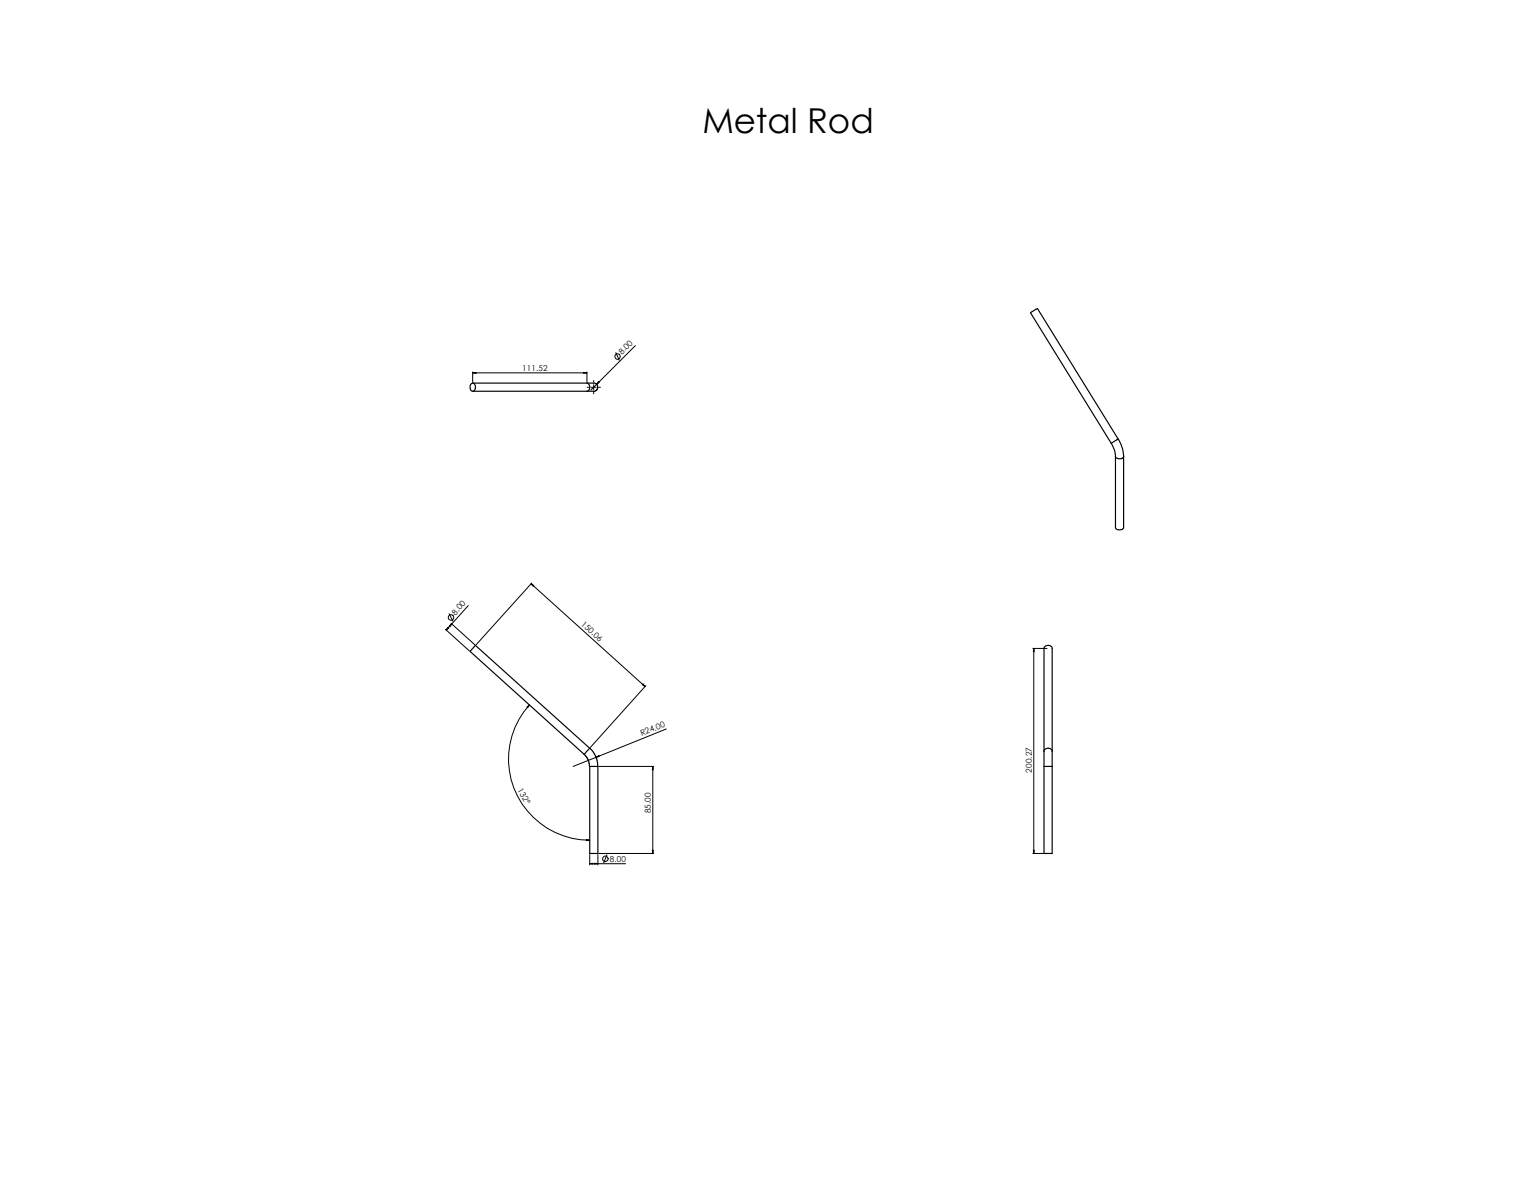
ISO-10303-21;
HEADER;
FILE_DESCRIPTION (('STEP AP214'),
    '1' );
FILE_NAME ('Metal Rod.step',
    '2026-10-20T14:49:59',
    ( '' ),
    ( '' ),
    'SwSTEP 2.0',
    'SolidWorks 2025',
    '' );
FILE_SCHEMA (( 'AUTOMOTIVE_DESIGN' ));
ENDSEC;

DATA;
#54=AXIS2_PLACEMENT_3D ( 'NONE', #4576, #604, #662 ) ;
#117=( NAMED_UNIT ( * ) SI_UNIT ( $, .STERADIAN. ) SOLID_ANGLE_UNIT ( ) );
#133=ADVANCED_BREP_SHAPE_REPRESENTATION ( '', ( #10321, #4601 ), #2278 ) ;
#147=SHAPE_REPRESENTATION_RELATIONSHIP ( 'NONE' , 'NONE' ,  #7587, #133 ) ;
#173=DIRECTION ( 'NONE',  ( 1.000000000000000000, 0.000000000000000000, 0.000000000000000000 ) ) ;
#205=CARTESIAN_POINT ( 'NONE',  ( -47.94539818030328604, 85.52895752738115220, 4.000000000000000000 ) ) ;
#218=VECTOR ( 'NONE', #1908, 1000.000000000000000 ) ;
#318=DIRECTION ( 'NONE',  ( 0.7431448254773962425, -0.6691306063588559061, 0.000000000000000000 ) ) ;
#324=DIRECTION ( 'NONE',  ( 6.106226635438360972E-16, -1.000000000000000000, 0.000000000000000000 ) ) ;
#334=ORIENTED_EDGE ( 'NONE', *, *, #6698, .T. ) ;
#338=CIRCLE ( 'NONE', #9475, 4.000000000000003553 ) ;
#367=DIRECTION ( 'NONE',  ( 1.000000000000000000, 0.000000000000000000, 0.000000000000000000 ) ) ;
#487=ADVANCED_FACE ( 'NONE', ( #1284 ), #6851, .T. ) ;
#497=CARTESIAN_POINT ( 'NONE',  ( -166.0794662972351716, 270.8019239353934040, 0.000000000000000000 ) ) ;
#536=ORIENTED_EDGE ( 'NONE', *, *, #7617, .T. ) ;
#601=CARTESIAN_POINT ( 'NONE',  ( -47.94539818030328604, 70.52895752738115220, 0.000000000000000000 ) ) ;
#604=DIRECTION ( 'NONE',  ( 0.000000000000000000, 0.000000000000000000, 1.000000000000000000 ) ) ;
#662=DIRECTION ( 'NONE',  ( 1.000000000000000000, 0.000000000000000000, 0.000000000000000000 ) ) ;
#682=CARTESIAN_POINT ( 'NONE',  ( -47.94539818030328604, 70.52895752738115220, -4.000000000000000000 ) ) ;
#741=ORIENTED_EDGE ( 'NONE', *, *, #7129, .T. ) ;
#749=CARTESIAN_POINT ( 'NONE',  ( -51.88626362769068123, 173.3644333388386940, 4.898587196589412829E-16 ) ) ;
#849=CARTESIAN_POINT ( 'NONE',  ( -166.0794662972351716, 270.8019239353934040, 0.000000000000000000 ) ) ;
#903=( NAMED_UNIT ( * ) PLANE_ANGLE_UNIT ( ) SI_UNIT ( $, .RADIAN. ) );
#922=DIRECTION ( 'NONE',  ( 0.000000000000000000, 1.000000000000000000, 0.000000000000000000 ) ) ;
#956=LINE ( 'NONE', #5088, #218 ) ;
#998=DIRECTION ( 'NONE',  ( 6.106226635438360972E-16, -1.000000000000000000, 0.000000000000000000 ) ) ;
#1070=DIRECTION ( 'NONE',  ( 1.000000000000000000, 0.000000000000000000, 0.000000000000000000 ) ) ;
#1154=DIRECTION ( 'NONE',  ( 0.000000000000000000, 1.000000000000000000, 0.000000000000000000 ) ) ;
#1284=FACE_OUTER_BOUND ( 'NONE', #3777, .T. ) ;
#1395=EDGE_CURVE ( 'NONE', #9655, #10447, #7716, .T. ) ;
#1528=DIRECTION ( 'NONE',  ( 1.000000000000000000, 0.000000000000000000, 0.000000000000000000 ) ) ;
#1635=AXIS2_PLACEMENT_3D ( 'NONE', #2392, #3294, #6585 ) ;
#1662=ORIENTED_EDGE ( 'NONE', *, *, #7675, .T. ) ;
#1863=CARTESIAN_POINT ( 'NONE',  ( -166.0794662972351716, 270.8019239353934040, 0.000000000000000000 ) ) ;
#1881=CIRCLE ( 'NONE', #54, 24.00000000000002132 ) ;
#1889=VERTEX_POINT ( 'NONE', #3894 ) ;
#1908=DIRECTION ( 'NONE',  ( -0.7431448254773957984, 0.6691306063588564612, 0.000000000000000000 ) ) ;
#1946=ORIENTED_EDGE ( 'NONE', *, *, #10327, .F. ) ;
#1950=DIRECTION ( 'NONE',  ( 1.000000000000000000, 6.106226635438360972E-16, 0.000000000000000000 ) ) ;
#2124=PRODUCT_DEFINITION_SHAPE ( 'NONE', 'NONE',  #3203 ) ;
#2211=DIRECTION ( 'NONE',  ( 0.7431448254773962425, -0.6691306063588559061, 0.000000000000000000 ) ) ;
#2214=CARTESIAN_POINT ( 'NONE',  ( -67.94539818030330025, 155.5289575273812090, 0.000000000000000000 ) ) ;
#2247=EDGE_CURVE ( 'NONE', #10447, #4228, #7356, .T. ) ;
#2278=( GEOMETRIC_REPRESENTATION_CONTEXT ( 3 ) GLOBAL_UNCERTAINTY_ASSIGNED_CONTEXT ( ( #3360 ) ) GLOBAL_UNIT_ASSIGNED_CONTEXT ( ( #7398, #6601, #9089 ) ) REPRESENTATION_CONTEXT ( 'NONE', 'WORKASPACE' ) );
#2317=AXIS2_PLACEMENT_3D ( 'NONE', #6483, #922, #7389 ) ;
#2320=ADVANCED_FACE ( 'NONE', ( #6609 ), #8357, .T. ) ;
#2340=EDGE_CURVE ( 'NONE', #10187, #1889, #5692, .T. ) ;
#2365=ORIENTED_EDGE ( 'NONE', *, *, #5529, .F. ) ;
#2392=CARTESIAN_POINT ( 'NONE',  ( -47.94539818030328604, 155.5289575273811522, 0.000000000000000000 ) ) ;
#2414=EDGE_CURVE ( 'NONE', #9655, #4137, #10114, .T. ) ;
#2441=DIRECTION ( 'NONE',  ( 0.6691306063588561281, 0.7431448254773961315, 0.000000000000000000 ) ) ;
#2460=ORIENTED_EDGE ( 'NONE', *, *, #2340, .F. ) ;
#2493=DIRECTION ( 'NONE',  ( 0.7431448254773962425, -0.6691306063588559061, 0.000000000000000000 ) ) ;
#2502=AXIS2_PLACEMENT_3D ( 'NONE', #7643, #3779, #4518 ) ;
#2585=CARTESIAN_POINT ( 'NONE',  ( -54.56278605312611774, 170.3918540369290895, 0.000000000000000000 ) ) ;
#2637=ORIENTED_EDGE ( 'NONE', *, *, #6913, .F. ) ;
#2676=ORIENTED_EDGE ( 'NONE', *, *, #7129, .F. ) ;
#2688=DIRECTION ( 'NONE',  ( -0.6691306063588561281, -0.7431448254773961315, 0.000000000000000000 ) ) ;
#2717=ORIENTED_EDGE ( 'NONE', *, *, #2340, .T. ) ;
#2745=AXIS2_PLACEMENT_3D ( 'NONE', #8570, #2211, #7779 ) ;
#2758=ORIENTED_EDGE ( 'NONE', *, *, #6627, .T. ) ;
#2982=PLANE ( 'NONE',  #3774 ) ;
#2997=AXIS2_PLACEMENT_3D ( 'NONE', #4334, #9858, #2688 ) ;
#3039=ORIENTED_EDGE ( 'NONE', *, *, #5529, .T. ) ;
#3095=CIRCLE ( 'NONE', #3428, 16.00000000000001421 ) ;
#3109=EDGE_CURVE ( 'NONE', #4228, #9114, #338, .T. ) ;
#3203=PRODUCT_DEFINITION ( 'UNKNOWN', '', #7860, #5677 ) ;
#3226=CARTESIAN_POINT ( 'NONE',  ( -47.94539818030328604, 155.5289575273811522, 4.000000000000000000 ) ) ;
#3234=( LENGTH_UNIT ( ) NAMED_UNIT ( * ) SI_UNIT ( .MILLI., .METRE. ) );
#3294=DIRECTION ( 'NONE',  ( 6.106226635438360972E-16, -1.000000000000000000, 0.000000000000000000 ) ) ;
#3360=UNCERTAINTY_MEASURE_WITH_UNIT (LENGTH_MEASURE( 1.000000000000000082E-05 ), #7398, 'distance_accuracy_value', 'NONE');
#3416=STYLED_ITEM('',(#10518),#10321);
#3422=CIRCLE ( 'NONE', #2745, 3.999999999999998668 ) ;
#3428=AXIS2_PLACEMENT_3D ( 'NONE', #9716, #7072, #9621 ) ;
#3444=ORIENTED_EDGE ( 'NONE', *, *, #2247, .F. ) ;
#3531=ORIENTED_EDGE ( 'NONE', *, *, #10340, .F. ) ;
#3546=CARTESIAN_POINT ( 'NONE',  ( -47.94539818030328604, 70.52895752738115220, 0.000000000000000000 ) ) ;
#3607=AXIS2_PLACEMENT_3D ( 'NONE', #9456, #5362, #5417 ) ;
#3700=CARTESIAN_POINT ( 'NONE',  ( -47.94539818030328604, 85.52895752738115220, -4.000000000000000000 ) ) ;
#3774=AXIS2_PLACEMENT_3D ( 'NONE', #497, #9346, #7859 ) ;
#3777=EDGE_LOOP ( 'NONE', ( #9685, #6029, #7830, #3039, #3444 ) ) ;
#3779=DIRECTION ( 'NONE',  ( 0.000000000000000000, 1.000000000000000000, 0.000000000000000000 ) ) ;
#3828=PRODUCT ( 'Metal Rod', 'Metal Rod', '', ( #10421 ) ) ;
#3851=VECTOR ( 'NONE', #1154, 1000.000000000000000 ) ;
#3894=CARTESIAN_POINT ( 'NONE',  ( -57.23930847856152582, 167.4192747350194850, 0.000000000000000000 ) ) ;
#3942=DIRECTION ( 'NONE',  ( 1.000000000000000000, 0.000000000000000000, 0.000000000000000000 ) ) ;
#4009=AXIS2_PLACEMENT_3D ( 'NONE', #1863, #5092, #8326 ) ;
#4111=TOROIDAL_SURFACE ( 'NONE', #3607, 20.00000000000001776, 4.000000000000000000 ) ;
#4137=VERTEX_POINT ( 'NONE', #4611 ) ;
#4149=AXIS2_PLACEMENT_3D ( 'NONE', #8366, #324, #1950 ) ;
#4228=VERTEX_POINT ( 'NONE', #3226 ) ;
#4312=CARTESIAN_POINT ( 'NONE',  ( -51.94539818030329315, 155.5289575273811522, -4.898587196589407898E-16 ) ) ;
#4334=CARTESIAN_POINT ( 'NONE',  ( -54.56278605312608931, 170.3918540369290895, 0.000000000000000000 ) ) ;
#4397=PLANE ( 'NONE',  #4149 ) ;
#4414=ADVANCED_FACE ( 'NONE', ( #8574 ), #4397, .T. ) ;
#4518=DIRECTION ( 'NONE',  ( 0.000000000000000000, 0.000000000000000000, 1.000000000000000000 ) ) ;
#4576=CARTESIAN_POINT ( 'NONE',  ( -67.94539818030330025, 155.5289575273812090, 0.000000000000000000 ) ) ;
#4601=AXIS2_PLACEMENT_3D ( 'NONE', #8586, #5983, #5928 ) ;
#4611=CARTESIAN_POINT ( 'NONE',  ( -47.94539818030328604, 155.5289575273811522, -4.000000000000000000 ) ) ;
#4614=ORIENTED_EDGE ( 'NONE', *, *, #10327, .T. ) ;
#4628=APPLICATION_CONTEXT ( 'automotive_design' ) ;
#4763=CIRCLE ( 'NONE', #5613, 4.000000000000003553 ) ;
#4815=ADVANCED_FACE ( 'NONE', ( #8137 ), #7349, .T. ) ;
#4891=CYLINDRICAL_SURFACE ( 'NONE', #2317, 4.000000000000000000 ) ;
#4931=ORIENTED_EDGE ( 'NONE', *, *, #7675, .F. ) ;
#5088=CARTESIAN_POINT ( 'NONE',  ( -57.23930847856151161, 167.4192747350194850, 0.000000000000000000 ) ) ;
#5092=DIRECTION ( 'NONE',  ( 0.7431448254773962425, -0.6691306063588559061, 0.000000000000000000 ) ) ;
#5094=DIRECTION ( 'NONE',  ( 6.106226635438360972E-16, -1.000000000000000000, 0.000000000000000000 ) ) ;
#5107=APPLICATION_CONTEXT ( 'automotive_design' ) ;
#5166=DIRECTION ( 'NONE',  ( -0.6691306063588561281, -0.7431448254773961315, 0.000000000000000000 ) ) ;
#5190=ADVANCED_FACE ( 'NONE', ( #9680 ), #4891, .T. ) ;
#5209=FACE_OUTER_BOUND ( 'NONE', #9931, .T. ) ;
#5210=CARTESIAN_POINT ( 'NONE',  ( -168.7559887226705655, 267.8293446334838563, 0.000000000000000000 ) ) ;
#5223=CARTESIAN_POINT ( 'NONE',  ( -54.56278605312608931, 170.3918540369290895, 0.000000000000000000 ) ) ;
#5302=VERTEX_POINT ( 'NONE', #5210 ) ;
#5362=DIRECTION ( 'NONE',  ( 0.000000000000000000, 0.000000000000000000, 1.000000000000000000 ) ) ;
#5368=CLOSED_SHELL ( 'NONE', ( #7444, #2320, #487, #4815, #8507, #5190, #7409, #4414 ) ) ;
#5412=ORIENTED_EDGE ( 'NONE', *, *, #6698, .F. ) ;
#5417=DIRECTION ( 'NONE',  ( 1.000000000000000000, 0.000000000000000000, 0.000000000000000000 ) ) ;
#5420=CARTESIAN_POINT ( 'NONE',  ( -51.88626362769066702, 173.3644333388386656, 4.898587196589412829E-16 ) ) ;
#5529=EDGE_CURVE ( 'NONE', #9125, #4228, #10282, .T. ) ;
#5613=AXIS2_PLACEMENT_3D ( 'NONE', #7428, #7474, #173 ) ;
#5657=CARTESIAN_POINT ( 'NONE',  ( -47.94539818030328604, 155.5289575273811522, 0.000000000000000000 ) ) ;
#5677=PRODUCT_DEFINITION_CONTEXT ( 'detailed design', #5107, 'design' ) ;
#5692=CIRCLE ( 'NONE', #6375, 3.999999999999998668 ) ;
#5725=EDGE_CURVE ( 'NONE', #9869, #5302, #8575, .T. ) ;
#5741=SHAPE_DEFINITION_REPRESENTATION ( #2124, #7587 ) ;
#5781=UNCERTAINTY_MEASURE_WITH_UNIT (LENGTH_MEASURE( 1.000000000000000082E-05 ), #3234, 'distance_accuracy_value', 'NONE');
#5888=CARTESIAN_POINT ( 'NONE',  ( -47.94539818030328604, 155.5289575273811522, 0.000000000000000000 ) ) ;
#5928=DIRECTION ( 'NONE',  ( 1.000000000000000000, 0.000000000000000000, 0.000000000000000000 ) ) ;
#5983=DIRECTION ( 'NONE',  ( 0.000000000000000000, 0.000000000000000000, 1.000000000000000000 ) ) ;
#6015=AXIS2_PLACEMENT_3D ( 'NONE', #3546, #6770, #367 ) ;
#6029=ORIENTED_EDGE ( 'NONE', *, *, #2414, .T. ) ;
#6153=ORIENTED_EDGE ( 'NONE', *, *, #6627, .F. ) ;
#6161=EDGE_LOOP ( 'NONE', ( #2460, #334, #7393, #4931 ) ) ;
#6296=AXIS2_PLACEMENT_3D ( 'NONE', #849, #2493, #2441 ) ;
#6329=EDGE_LOOP ( 'NONE', ( #5412, #2676, #1662, #6904 ) ) ;
#6334=AXIS2_PLACEMENT_3D ( 'NONE', #2214, #10227, #1528 ) ;
#6374=LINE ( 'NONE', #5420, #9686 ) ;
#6375=AXIS2_PLACEMENT_3D ( 'NONE', #2585, #318, #9103 ) ;
#6464=ORIENTED_EDGE ( 'NONE', *, *, #7617, .F. ) ;
#6483=CARTESIAN_POINT ( 'NONE',  ( -47.94539818030328604, 85.52895752738115220, 0.000000000000000000 ) ) ;
#6585=DIRECTION ( 'NONE',  ( 1.000000000000000000, 0.000000000000000000, 0.000000000000000000 ) ) ;
#6601=( NAMED_UNIT ( * ) PLANE_ANGLE_UNIT ( ) SI_UNIT ( $, .RADIAN. ) );
#6609=FACE_OUTER_BOUND ( 'NONE', #6161, .T. ) ;
#6624=AXIS2_PLACEMENT_3D ( 'NONE', #5657, #998, #8146 ) ;
#6627=EDGE_CURVE ( 'NONE', #9125, #10187, #1881, .T. ) ;
#6698=EDGE_CURVE ( 'NONE', #10187, #9869, #6374, .T. ) ;
#6717=VECTOR ( 'NONE', #8996, 1000.000000000000000 ) ;
#6770=DIRECTION ( 'NONE',  ( 6.106226635438360972E-16, -1.000000000000000000, 0.000000000000000000 ) ) ;
#6851=CYLINDRICAL_SURFACE ( 'NONE', #2502, 4.000000000000000000 ) ;
#6863=AXIS2_PLACEMENT_3D ( 'NONE', #5223, #8506, #5166 ) ;
#6904=ORIENTED_EDGE ( 'NONE', *, *, #10340, .T. ) ;
#6913=EDGE_CURVE ( 'NONE', #4137, #9125, #7143, .T. ) ;
#6973=MECHANICAL_DESIGN_GEOMETRIC_PRESENTATION_REPRESENTATION('',(#3416),#9687);
#7072=DIRECTION ( 'NONE',  ( 0.000000000000000000, 0.000000000000000000, 1.000000000000000000 ) ) ;
#7129=EDGE_CURVE ( 'NONE', #1889, #10187, #3422, .T. ) ;
#7143=CIRCLE ( 'NONE', #6624, 4.000000000000003553 ) ;
#7156=ORIENTED_EDGE ( 'NONE', *, *, #5725, .F. ) ;
#7243=ORIENTED_EDGE ( 'NONE', *, *, #2414, .F. ) ;
#7349=CYLINDRICAL_SURFACE ( 'NONE', #6863, 3.999999999999998668 ) ;
#7356=LINE ( 'NONE', #205, #6717 ) ;
#7389=DIRECTION ( 'NONE',  ( 0.000000000000000000, 0.000000000000000000, 1.000000000000000000 ) ) ;
#7393=ORIENTED_EDGE ( 'NONE', *, *, #5725, .T. ) ;
#7398=( LENGTH_UNIT ( ) NAMED_UNIT ( * ) SI_UNIT ( .MILLI., .METRE. ) );
#7409=ADVANCED_FACE ( 'NONE', ( #9296 ), #2982, .F. ) ;
#7428=CARTESIAN_POINT ( 'NONE',  ( -47.94539818030328604, 155.5289575273811522, 0.000000000000000000 ) ) ;
#7444=ADVANCED_FACE ( 'NONE', ( #5209 ), #4111, .T. ) ;
#7449=ORIENTED_EDGE ( 'NONE', *, *, #3109, .T. ) ;
#7474=DIRECTION ( 'NONE',  ( 6.106226635438360972E-16, -1.000000000000000000, 0.000000000000000000 ) ) ;
#7476=CIRCLE ( 'NONE', #6296, 3.999999999999998668 ) ;
#7538=EDGE_CURVE ( 'NONE', #10447, #9655, #10207, .T. ) ;
#7587=SHAPE_REPRESENTATION ( 'Metal Rod', ( #4601 ), #2278 ) ;
#7617=EDGE_CURVE ( 'NONE', #9114, #1889, #3095, .T. ) ;
#7643=CARTESIAN_POINT ( 'NONE',  ( -47.94539818030328604, 85.52895752738115220, 0.000000000000000000 ) ) ;
#7675=EDGE_CURVE ( 'NONE', #1889, #5302, #956, .T. ) ;
#7688=CARTESIAN_POINT ( 'NONE',  ( -47.94539818030328604, 70.52895752738115220, 4.000000000000000000 ) ) ;
#7694=EDGE_LOOP ( 'NONE', ( #3531, #7156 ) ) ;
#7716=CIRCLE ( 'NONE', #6015, 4.000000000000003553 ) ;
#7745=CARTESIAN_POINT ( 'NONE',  ( -43.94539818030328604, 155.5289575273811522, 0.000000000000000000 ) ) ;
#7779=DIRECTION ( 'NONE',  ( 0.6691306063588561281, 0.7431448254773961315, 0.000000000000000000 ) ) ;
#7830=ORIENTED_EDGE ( 'NONE', *, *, #6913, .T. ) ;
#7859=DIRECTION ( 'NONE',  ( 0.6691306063588559061, 0.7431448254773963535, 0.000000000000000000 ) ) ;
#7860=PRODUCT_DEFINITION_FORMATION_WITH_SPECIFIED_SOURCE ( 'ANY', '', #3828, .NOT_KNOWN. ) ;
#8137=FACE_OUTER_BOUND ( 'NONE', #6329, .T. ) ;
#8146=DIRECTION ( 'NONE',  ( 1.000000000000000000, 0.000000000000000000, 0.000000000000000000 ) ) ;
#8157=ORIENTED_EDGE ( 'NONE', *, *, #7538, .F. ) ;
#8326=DIRECTION ( 'NONE',  ( 0.6691306063588561281, 0.7431448254773961315, 0.000000000000000000 ) ) ;
#8357=CYLINDRICAL_SURFACE ( 'NONE', #2997, 3.999999999999998668 ) ;
#8366=CARTESIAN_POINT ( 'NONE',  ( -47.94539818030327893, 70.52895752738115220, 0.000000000000000000 ) ) ;
#8472=EDGE_LOOP ( 'NONE', ( #10160, #8804 ) ) ;
#8506=DIRECTION ( 'NONE',  ( -0.7431448254773957984, 0.6691306063588564612, 0.000000000000000000 ) ) ;
#8507=ADVANCED_FACE ( 'NONE', ( #9429 ), #8866, .T. ) ;
#8509=CARTESIAN_POINT ( 'NONE',  ( -163.4029438717997209, 273.7745032373030085, 4.898587196589412829E-16 ) ) ;
#8570=CARTESIAN_POINT ( 'NONE',  ( -54.56278605312611774, 170.3918540369290895, 0.000000000000000000 ) ) ;
#8574=FACE_OUTER_BOUND ( 'NONE', #8472, .T. ) ;
#8575=CIRCLE ( 'NONE', #4009, 3.999999999999998668 ) ;
#8586=CARTESIAN_POINT ( 'NONE',  ( 0.000000000000000000, 0.000000000000000000, 0.000000000000000000 ) ) ;
#8606=DIRECTION ( 'NONE',  ( -0.7431448254773957984, 0.6691306063588564612, 0.000000000000000000 ) ) ;
#8760=DIRECTION ( 'NONE',  ( 6.106226635438360972E-16, -1.000000000000000000, 0.000000000000000000 ) ) ;
#8804=ORIENTED_EDGE ( 'NONE', *, *, #1395, .T. ) ;
#8866=TOROIDAL_SURFACE ( 'NONE', #6334, 20.00000000000001776, 4.000000000000000000 ) ;
#8996=DIRECTION ( 'NONE',  ( 0.000000000000000000, 1.000000000000000000, 0.000000000000000000 ) ) ;
#9089=( NAMED_UNIT ( * ) SI_UNIT ( $, .STERADIAN. ) SOLID_ANGLE_UNIT ( ) );
#9103=DIRECTION ( 'NONE',  ( 0.6691306063588561281, 0.7431448254773961315, 0.000000000000000000 ) ) ;
#9114=VERTEX_POINT ( 'NONE', #4312 ) ;
#9125=VERTEX_POINT ( 'NONE', #7745 ) ;
#9296=FACE_OUTER_BOUND ( 'NONE', #7694, .T. ) ;
#9346=DIRECTION ( 'NONE',  ( 0.7431448254773963535, -0.6691306063588559061, 0.000000000000000000 ) ) ;
#9429=FACE_OUTER_BOUND ( 'NONE', #10316, .T. ) ;
#9456=CARTESIAN_POINT ( 'NONE',  ( -67.94539818030330025, 155.5289575273812090, 0.000000000000000000 ) ) ;
#9475=AXIS2_PLACEMENT_3D ( 'NONE', #5888, #5094, #1070 ) ;
#9621=DIRECTION ( 'NONE',  ( 1.000000000000000000, 0.000000000000000000, 0.000000000000000000 ) ) ;
#9655=VERTEX_POINT ( 'NONE', #682 ) ;
#9680=FACE_OUTER_BOUND ( 'NONE', #10170, .T. ) ;
#9685=ORIENTED_EDGE ( 'NONE', *, *, #1395, .F. ) ;
#9686=VECTOR ( 'NONE', #8606, 1000.000000000000000 ) ;
#9687=( GEOMETRIC_REPRESENTATION_CONTEXT ( 3 ) GLOBAL_UNCERTAINTY_ASSIGNED_CONTEXT ( ( #5781 ) ) GLOBAL_UNIT_ASSIGNED_CONTEXT ( ( #3234, #903, #117 ) ) REPRESENTATION_CONTEXT ( 'NONE', 'WORKASPACE' ) );
#9700=ORIENTED_EDGE ( 'NONE', *, *, #3109, .F. ) ;
#9716=CARTESIAN_POINT ( 'NONE',  ( -67.94539818030330025, 155.5289575273812090, -4.898587196589412829E-16 ) ) ;
#9858=DIRECTION ( 'NONE',  ( -0.7431448254773957984, 0.6691306063588564612, 0.000000000000000000 ) ) ;
#9869=VERTEX_POINT ( 'NONE', #8509 ) ;
#9931=EDGE_LOOP ( 'NONE', ( #2365, #2758, #2717, #6464, #9700 ) ) ;
#9985=ORIENTED_EDGE ( 'NONE', *, *, #2247, .T. ) ;
#10038=AXIS2_PLACEMENT_3D ( 'NONE', #601, #8760, #3942 ) ;
#10114=LINE ( 'NONE', #3700, #3851 ) ;
#10160=ORIENTED_EDGE ( 'NONE', *, *, #7538, .T. ) ;
#10170=EDGE_LOOP ( 'NONE', ( #7243, #8157, #9985, #7449, #4614 ) ) ;
#10187=VERTEX_POINT ( 'NONE', #749 ) ;
#10207=CIRCLE ( 'NONE', #10038, 4.000000000000003553 ) ;
#10227=DIRECTION ( 'NONE',  ( 0.000000000000000000, 0.000000000000000000, 1.000000000000000000 ) ) ;
#10282=CIRCLE ( 'NONE', #1635, 4.000000000000003553 ) ;
#10316=EDGE_LOOP ( 'NONE', ( #6153, #2637, #1946, #536, #741 ) ) ;
#10321=MANIFOLD_SOLID_BREP ( 'Move Face3', #5368 ) ;
#10327=EDGE_CURVE ( 'NONE', #9114, #4137, #4763, .T. ) ;
#10340=EDGE_CURVE ( 'NONE', #5302, #9869, #7476, .T. ) ;
#10421=PRODUCT_CONTEXT ( 'NONE', #4628, 'mechanical' ) ;
#10447=VERTEX_POINT ( 'NONE', #7688 ) ;
#10512=COLOUR_RGB('Grey',0.48,0.52,0.57);
#10513=FILL_AREA_STYLE_COLOUR('',#10512);
#10514=FILL_AREA_STYLE('',(#10513));
#10515=SURFACE_STYLE_FILL_AREA(#10514);
#10516=SURFACE_SIDE_STYLE('',(#10515));
#10517=SURFACE_STYLE_USAGE(.BOTH.,#10516);
#10518=PRESENTATION_STYLE_ASSIGNMENT((#10517));
ENDSEC;
END-ISO-10303-21;
